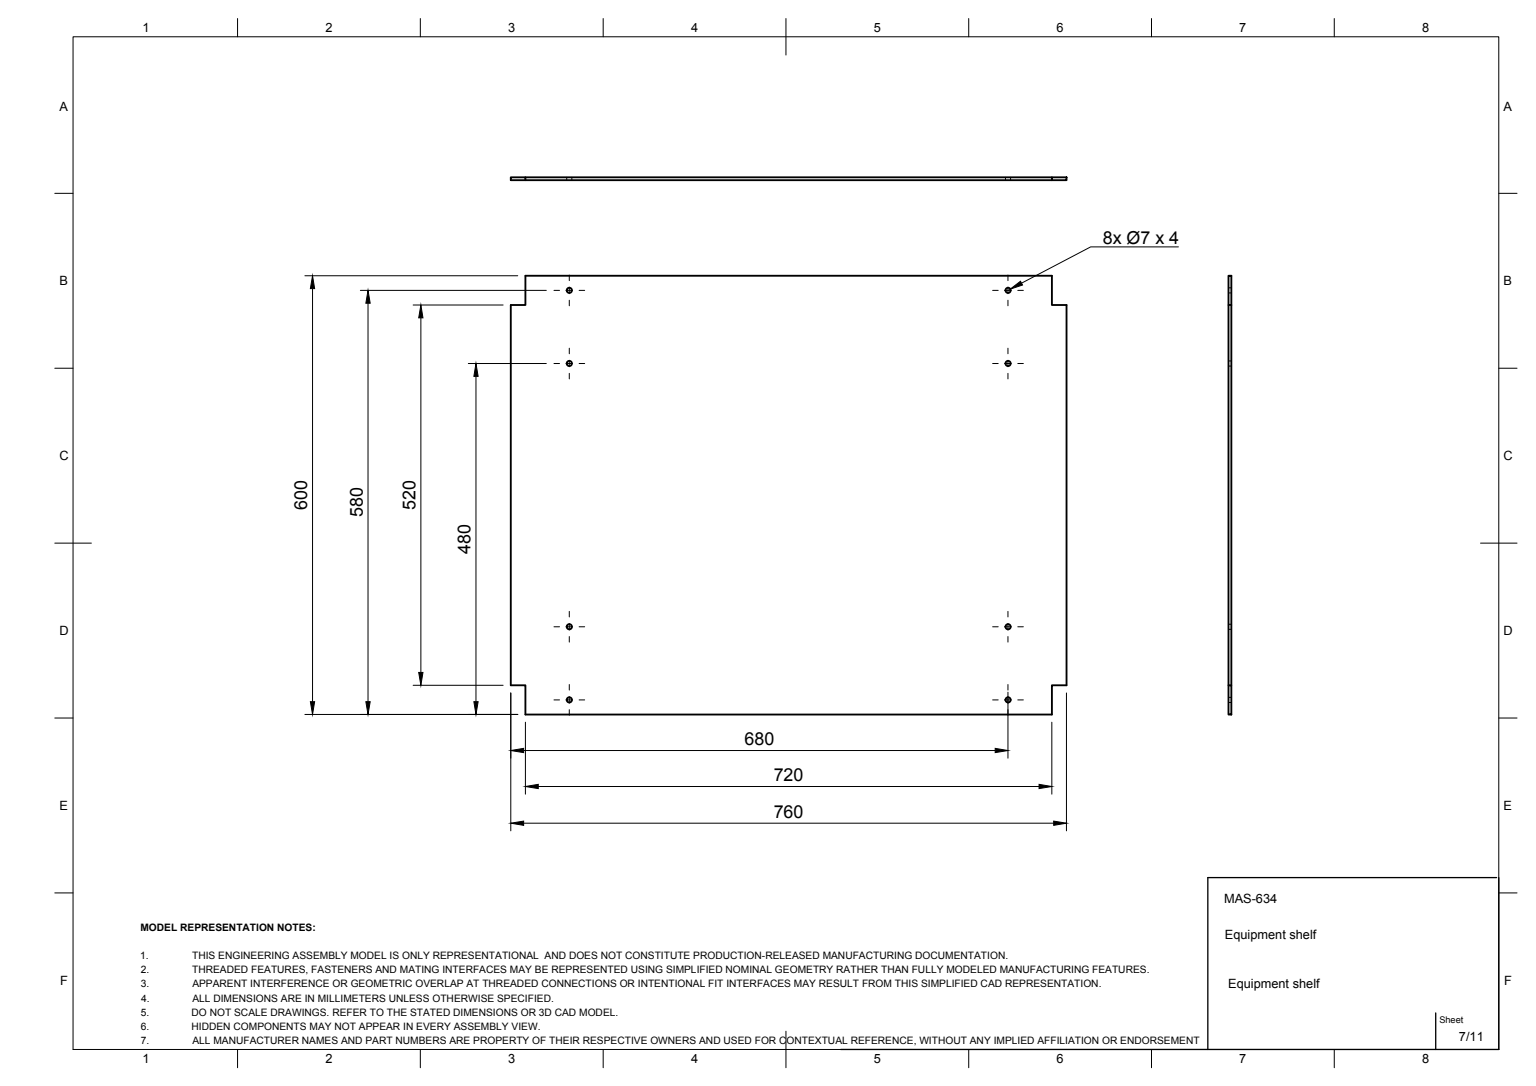
ISO-10303-21;
HEADER;
/* Generated by software containing ST-Developer
 * from STEP Tools, Inc. (www.steptools.com) 
 */

FILE_DESCRIPTION(
/* description */ ('Independent AHU equipment rack. Nominal800x600 frame on1000long40squa
re aluminum posts; two removable notched shelves; welded perimeter/cro
ss rails and rear gussets; two mounting channels; four isolation pads 
and anchor-ready feet. Imported native extrusion library retained and 
cut-length parameters customized per family. Shelf hardware uses model
ed M6 rivet nuts and screws. Weld design, floor anchors and load ratin
g require engineering selection.'),
/* implementation_level */ '2;1');

FILE_NAME(
/* name */ 'Equipment shelf.step',
/* time_stamp */ '2026-11-07T19:04:45-08:00',
/* author */ (''),
/* organization */ (''),
/* preprocessor_version */ 'ST-DEVELOPER v20.2',
/* originating_system */ 'Autodesk Translation Framework v15.17.0.0',
/* authorisation */ '');

FILE_SCHEMA (('AUTOMOTIVE_DESIGN { 1 0 10303 214 3 1 1 }'));
ENDSEC;

DATA;
#10=MECHANICAL_DESIGN_GEOMETRIC_PRESENTATION_REPRESENTATION('',(#339),#9777);
#317=SHAPE_REPRESENTATION_RELATIONSHIP('SRR','None',#9861,#328);
#328=ADVANCED_BREP_SHAPE_REPRESENTATION('',(#350),#9770);
#339=STYLED_ITEM('',(#9924),#350);
#350=MANIFOLD_SOLID_BREP('Body1',#3844);
#371=FACE_BOUND('',#809,.T.);
#372=FACE_BOUND('',#810,.T.);
#373=FACE_BOUND('',#811,.T.);
#374=FACE_BOUND('',#812,.T.);
#375=FACE_BOUND('',#813,.T.);
#376=FACE_BOUND('',#814,.T.);
#377=FACE_BOUND('',#815,.T.);
#378=FACE_BOUND('',#816,.T.);
#379=FACE_BOUND('',#818,.T.);
#380=FACE_BOUND('',#819,.T.);
#381=FACE_BOUND('',#820,.T.);
#382=FACE_BOUND('',#821,.T.);
#383=FACE_BOUND('',#822,.T.);
#384=FACE_BOUND('',#823,.T.);
#385=FACE_BOUND('',#824,.T.);
#386=FACE_BOUND('',#825,.T.);
#450=PLANE('',#4151);
#451=PLANE('',#4152);
#452=PLANE('',#4153);
#453=PLANE('',#4154);
#454=PLANE('',#4155);
#455=PLANE('',#4156);
#456=PLANE('',#4157);
#457=PLANE('',#4158);
#458=PLANE('',#4159);
#459=PLANE('',#4160);
#460=PLANE('',#4161);
#461=PLANE('',#4162);
#462=PLANE('',#4163);
#463=PLANE('',#4164);
#578=FACE_OUTER_BOUND('',#790,.T.);
#579=FACE_OUTER_BOUND('',#791,.T.);
#580=FACE_OUTER_BOUND('',#792,.T.);
#581=FACE_OUTER_BOUND('',#793,.T.);
#582=FACE_OUTER_BOUND('',#794,.T.);
#583=FACE_OUTER_BOUND('',#795,.T.);
#584=FACE_OUTER_BOUND('',#796,.T.);
#585=FACE_OUTER_BOUND('',#797,.T.);
#586=FACE_OUTER_BOUND('',#798,.T.);
#587=FACE_OUTER_BOUND('',#799,.T.);
#588=FACE_OUTER_BOUND('',#800,.T.);
#589=FACE_OUTER_BOUND('',#801,.T.);
#590=FACE_OUTER_BOUND('',#802,.T.);
#591=FACE_OUTER_BOUND('',#803,.T.);
#592=FACE_OUTER_BOUND('',#804,.T.);
#593=FACE_OUTER_BOUND('',#805,.T.);
#594=FACE_OUTER_BOUND('',#806,.T.);
#595=FACE_OUTER_BOUND('',#807,.T.);
#596=FACE_OUTER_BOUND('',#808,.T.);
#597=FACE_OUTER_BOUND('',#817,.T.);
#598=FACE_OUTER_BOUND('',#826,.T.);
#599=FACE_OUTER_BOUND('',#827,.T.);
#790=EDGE_LOOP('',(#2923,#2924,#2925,#2926));
#791=EDGE_LOOP('',(#2927,#2928,#2929,#2930));
#792=EDGE_LOOP('',(#2931,#2932,#2933,#2934));
#793=EDGE_LOOP('',(#2935,#2936,#2937,#2938));
#794=EDGE_LOOP('',(#2939,#2940,#2941,#2942));
#795=EDGE_LOOP('',(#2943,#2944,#2945,#2946));
#796=EDGE_LOOP('',(#2947,#2948,#2949,#2950));
#797=EDGE_LOOP('',(#2951,#2952,#2953,#2954));
#798=EDGE_LOOP('',(#2955,#2956,#2957,#2958));
#799=EDGE_LOOP('',(#2959,#2960,#2961,#2962));
#800=EDGE_LOOP('',(#2963,#2964,#2965,#2966));
#801=EDGE_LOOP('',(#2967,#2968,#2969,#2970));
#802=EDGE_LOOP('',(#2971,#2972,#2973,#2974));
#803=EDGE_LOOP('',(#2975,#2976,#2977,#2978));
#804=EDGE_LOOP('',(#2979,#2980,#2981,#2982));
#805=EDGE_LOOP('',(#2983,#2984,#2985,#2986));
#806=EDGE_LOOP('',(#2987,#2988,#2989,#2990));
#807=EDGE_LOOP('',(#2991,#2992,#2993,#2994));
#808=EDGE_LOOP('',(#2995,#2996,#2997,#2998,#2999,#3000,#3001,#3002,#3003,
#3004,#3005,#3006));
#809=EDGE_LOOP('',(#3007));
#810=EDGE_LOOP('',(#3008));
#811=EDGE_LOOP('',(#3009));
#812=EDGE_LOOP('',(#3010));
#813=EDGE_LOOP('',(#3011));
#814=EDGE_LOOP('',(#3012));
#815=EDGE_LOOP('',(#3013));
#816=EDGE_LOOP('',(#3014));
#817=EDGE_LOOP('',(#3015,#3016,#3017,#3018,#3019,#3020,#3021,#3022,#3023,
#3024,#3025,#3026));
#818=EDGE_LOOP('',(#3027));
#819=EDGE_LOOP('',(#3028));
#820=EDGE_LOOP('',(#3029));
#821=EDGE_LOOP('',(#3030));
#822=EDGE_LOOP('',(#3031));
#823=EDGE_LOOP('',(#3032));
#824=EDGE_LOOP('',(#3033));
#825=EDGE_LOOP('',(#3034));
#826=EDGE_LOOP('',(#3035,#3036,#3037,#3038));
#827=EDGE_LOOP('',(#3039,#3040,#3041,#3042));
#1083=LINE('',#5829,#1376);
#1084=LINE('',#5835,#1377);
#1085=LINE('',#5841,#1378);
#1086=LINE('',#5847,#1379);
#1087=LINE('',#5853,#1380);
#1088=LINE('',#5859,#1381);
#1089=LINE('',#5865,#1382);
#1090=LINE('',#5871,#1383);
#1091=LINE('',#5876,#1384);
#1092=LINE('',#5878,#1385);
#1093=LINE('',#5880,#1386);
#1094=LINE('',#5881,#1387);
#1095=LINE('',#5884,#1388);
#1096=LINE('',#5886,#1389);
#1097=LINE('',#5887,#1390);
#1098=LINE('',#5891,#1391);
#1099=LINE('',#5893,#1392);
#1100=LINE('',#5895,#1393);
#1101=LINE('',#5896,#1394);
#1102=LINE('',#5899,#1395);
#1103=LINE('',#5901,#1396);
#1104=LINE('',#5902,#1397);
#1105=LINE('',#5906,#1398);
#1106=LINE('',#5908,#1399);
#1107=LINE('',#5910,#1400);
#1108=LINE('',#5911,#1401);
#1109=LINE('',#5914,#1402);
#1110=LINE('',#5916,#1403);
#1111=LINE('',#5917,#1404);
#1112=LINE('',#5921,#1405);
#1113=LINE('',#5923,#1406);
#1114=LINE('',#5925,#1407);
#1115=LINE('',#5926,#1408);
#1116=LINE('',#5929,#1409);
#1117=LINE('',#5931,#1410);
#1118=LINE('',#5932,#1411);
#1119=LINE('',#5934,#1412);
#1120=LINE('',#5935,#1413);
#1121=LINE('',#5937,#1414);
#1122=LINE('',#5938,#1415);
#1123=LINE('',#5940,#1416);
#1124=LINE('',#5941,#1417);
#1125=LINE('',#5943,#1418);
#1126=LINE('',#5944,#1419);
#1376=VECTOR('',#4796,3.5);
#1377=VECTOR('',#4803,3.5);
#1378=VECTOR('',#4810,3.5);
#1379=VECTOR('',#4817,3.5);
#1380=VECTOR('',#4824,3.5);
#1381=VECTOR('',#4831,3.5);
#1382=VECTOR('',#4838,3.5);
#1383=VECTOR('',#4845,3.5);
#1384=VECTOR('',#4850,10.);
#1385=VECTOR('',#4851,10.);
#1386=VECTOR('',#4852,10.);
#1387=VECTOR('',#4853,10.);
#1388=VECTOR('',#4856,10.);
#1389=VECTOR('',#4857,10.);
#1390=VECTOR('',#4858,10.);
#1391=VECTOR('',#4861,10.);
#1392=VECTOR('',#4862,10.);
#1393=VECTOR('',#4863,10.);
#1394=VECTOR('',#4864,10.);
#1395=VECTOR('',#4867,10.);
#1396=VECTOR('',#4868,10.);
#1397=VECTOR('',#4869,10.);
#1398=VECTOR('',#4872,10.);
#1399=VECTOR('',#4873,10.);
#1400=VECTOR('',#4874,10.);
#1401=VECTOR('',#4875,10.);
#1402=VECTOR('',#4878,10.);
#1403=VECTOR('',#4879,10.);
#1404=VECTOR('',#4880,10.);
#1405=VECTOR('',#4883,10.);
#1406=VECTOR('',#4884,10.);
#1407=VECTOR('',#4885,10.);
#1408=VECTOR('',#4886,10.);
#1409=VECTOR('',#4889,10.);
#1410=VECTOR('',#4890,10.);
#1411=VECTOR('',#4891,10.);
#1412=VECTOR('',#4894,10.);
#1413=VECTOR('',#4895,10.);
#1414=VECTOR('',#4898,10.);
#1415=VECTOR('',#4899,10.);
#1416=VECTOR('',#4902,10.);
#1417=VECTOR('',#4903,10.);
#1418=VECTOR('',#4906,10.);
#1419=VECTOR('',#4907,10.);
#1609=CIRCLE('',#4128,3.5);
#1610=CIRCLE('',#4129,3.5);
#1611=CIRCLE('',#4131,3.5);
#1612=CIRCLE('',#4132,3.5);
#1613=CIRCLE('',#4134,3.5);
#1614=CIRCLE('',#4135,3.5);
#1615=CIRCLE('',#4137,3.5);
#1616=CIRCLE('',#4138,3.5);
#1617=CIRCLE('',#4140,3.5);
#1618=CIRCLE('',#4141,3.5);
#1619=CIRCLE('',#4143,3.5);
#1620=CIRCLE('',#4144,3.5);
#1621=CIRCLE('',#4146,3.5);
#1622=CIRCLE('',#4147,3.5);
#1623=CIRCLE('',#4149,3.5);
#1624=CIRCLE('',#4150,3.5);
#1796=VERTEX_POINT('',#5826);
#1797=VERTEX_POINT('',#5828);
#1798=VERTEX_POINT('',#5832);
#1799=VERTEX_POINT('',#5834);
#1800=VERTEX_POINT('',#5838);
#1801=VERTEX_POINT('',#5840);
#1802=VERTEX_POINT('',#5844);
#1803=VERTEX_POINT('',#5846);
#1804=VERTEX_POINT('',#5850);
#1805=VERTEX_POINT('',#5852);
#1806=VERTEX_POINT('',#5856);
#1807=VERTEX_POINT('',#5858);
#1808=VERTEX_POINT('',#5862);
#1809=VERTEX_POINT('',#5864);
#1810=VERTEX_POINT('',#5868);
#1811=VERTEX_POINT('',#5870);
#1812=VERTEX_POINT('',#5874);
#1813=VERTEX_POINT('',#5875);
#1814=VERTEX_POINT('',#5877);
#1815=VERTEX_POINT('',#5879);
#1816=VERTEX_POINT('',#5883);
#1817=VERTEX_POINT('',#5885);
#1818=VERTEX_POINT('',#5889);
#1819=VERTEX_POINT('',#5890);
#1820=VERTEX_POINT('',#5892);
#1821=VERTEX_POINT('',#5894);
#1822=VERTEX_POINT('',#5898);
#1823=VERTEX_POINT('',#5900);
#1824=VERTEX_POINT('',#5904);
#1825=VERTEX_POINT('',#5905);
#1826=VERTEX_POINT('',#5907);
#1827=VERTEX_POINT('',#5909);
#1828=VERTEX_POINT('',#5913);
#1829=VERTEX_POINT('',#5915);
#1830=VERTEX_POINT('',#5919);
#1831=VERTEX_POINT('',#5920);
#1832=VERTEX_POINT('',#5922);
#1833=VERTEX_POINT('',#5924);
#1834=VERTEX_POINT('',#5928);
#1835=VERTEX_POINT('',#5930);
#2206=EDGE_CURVE('',#1796,#1796,#1609,.T.);
#2207=EDGE_CURVE('',#1796,#1797,#1083,.T.);
#2208=EDGE_CURVE('',#1797,#1797,#1610,.T.);
#2209=EDGE_CURVE('',#1798,#1798,#1611,.T.);
#2210=EDGE_CURVE('',#1798,#1799,#1084,.T.);
#2211=EDGE_CURVE('',#1799,#1799,#1612,.T.);
#2212=EDGE_CURVE('',#1800,#1800,#1613,.T.);
#2213=EDGE_CURVE('',#1800,#1801,#1085,.T.);
#2214=EDGE_CURVE('',#1801,#1801,#1614,.T.);
#2215=EDGE_CURVE('',#1802,#1802,#1615,.T.);
#2216=EDGE_CURVE('',#1802,#1803,#1086,.T.);
#2217=EDGE_CURVE('',#1803,#1803,#1616,.T.);
#2218=EDGE_CURVE('',#1804,#1804,#1617,.T.);
#2219=EDGE_CURVE('',#1804,#1805,#1087,.T.);
#2220=EDGE_CURVE('',#1805,#1805,#1618,.T.);
#2221=EDGE_CURVE('',#1806,#1806,#1619,.T.);
#2222=EDGE_CURVE('',#1806,#1807,#1088,.T.);
#2223=EDGE_CURVE('',#1807,#1807,#1620,.T.);
#2224=EDGE_CURVE('',#1808,#1808,#1621,.T.);
#2225=EDGE_CURVE('',#1808,#1809,#1089,.T.);
#2226=EDGE_CURVE('',#1809,#1809,#1622,.T.);
#2227=EDGE_CURVE('',#1810,#1810,#1623,.T.);
#2228=EDGE_CURVE('',#1810,#1811,#1090,.T.);
#2229=EDGE_CURVE('',#1811,#1811,#1624,.T.);
#2230=EDGE_CURVE('',#1812,#1813,#1091,.T.);
#2231=EDGE_CURVE('',#1812,#1814,#1092,.T.);
#2232=EDGE_CURVE('',#1815,#1814,#1093,.T.);
#2233=EDGE_CURVE('',#1813,#1815,#1094,.T.);
#2234=EDGE_CURVE('',#1816,#1812,#1095,.T.);
#2235=EDGE_CURVE('',#1817,#1816,#1096,.T.);
#2236=EDGE_CURVE('',#1814,#1817,#1097,.T.);
#2237=EDGE_CURVE('',#1818,#1819,#1098,.T.);
#2238=EDGE_CURVE('',#1818,#1820,#1099,.T.);
#2239=EDGE_CURVE('',#1821,#1820,#1100,.T.);
#2240=EDGE_CURVE('',#1819,#1821,#1101,.T.);
#2241=EDGE_CURVE('',#1822,#1818,#1102,.T.);
#2242=EDGE_CURVE('',#1823,#1822,#1103,.T.);
#2243=EDGE_CURVE('',#1820,#1823,#1104,.T.);
#2244=EDGE_CURVE('',#1824,#1825,#1105,.T.);
#2245=EDGE_CURVE('',#1824,#1826,#1106,.T.);
#2246=EDGE_CURVE('',#1827,#1826,#1107,.T.);
#2247=EDGE_CURVE('',#1825,#1827,#1108,.T.);
#2248=EDGE_CURVE('',#1828,#1824,#1109,.T.);
#2249=EDGE_CURVE('',#1829,#1828,#1110,.T.);
#2250=EDGE_CURVE('',#1826,#1829,#1111,.T.);
#2251=EDGE_CURVE('',#1830,#1831,#1112,.T.);
#2252=EDGE_CURVE('',#1832,#1830,#1113,.T.);
#2253=EDGE_CURVE('',#1833,#1832,#1114,.T.);
#2254=EDGE_CURVE('',#1831,#1833,#1115,.T.);
#2255=EDGE_CURVE('',#1831,#1834,#1116,.T.);
#2256=EDGE_CURVE('',#1835,#1833,#1117,.T.);
#2257=EDGE_CURVE('',#1834,#1835,#1118,.T.);
#2258=EDGE_CURVE('',#1821,#1829,#1119,.T.);
#2259=EDGE_CURVE('',#1819,#1828,#1120,.T.);
#2260=EDGE_CURVE('',#1834,#1822,#1121,.T.);
#2261=EDGE_CURVE('',#1835,#1823,#1122,.T.);
#2262=EDGE_CURVE('',#1827,#1817,#1123,.T.);
#2263=EDGE_CURVE('',#1815,#1832,#1124,.T.);
#2264=EDGE_CURVE('',#1813,#1830,#1125,.T.);
#2265=EDGE_CURVE('',#1825,#1816,#1126,.T.);
#2923=ORIENTED_EDGE('',*,*,#2206,.F.);
#2924=ORIENTED_EDGE('',*,*,#2207,.T.);
#2925=ORIENTED_EDGE('',*,*,#2208,.F.);
#2926=ORIENTED_EDGE('',*,*,#2207,.F.);
#2927=ORIENTED_EDGE('',*,*,#2209,.F.);
#2928=ORIENTED_EDGE('',*,*,#2210,.T.);
#2929=ORIENTED_EDGE('',*,*,#2211,.F.);
#2930=ORIENTED_EDGE('',*,*,#2210,.F.);
#2931=ORIENTED_EDGE('',*,*,#2212,.F.);
#2932=ORIENTED_EDGE('',*,*,#2213,.T.);
#2933=ORIENTED_EDGE('',*,*,#2214,.F.);
#2934=ORIENTED_EDGE('',*,*,#2213,.F.);
#2935=ORIENTED_EDGE('',*,*,#2215,.F.);
#2936=ORIENTED_EDGE('',*,*,#2216,.T.);
#2937=ORIENTED_EDGE('',*,*,#2217,.F.);
#2938=ORIENTED_EDGE('',*,*,#2216,.F.);
#2939=ORIENTED_EDGE('',*,*,#2218,.F.);
#2940=ORIENTED_EDGE('',*,*,#2219,.T.);
#2941=ORIENTED_EDGE('',*,*,#2220,.F.);
#2942=ORIENTED_EDGE('',*,*,#2219,.F.);
#2943=ORIENTED_EDGE('',*,*,#2221,.F.);
#2944=ORIENTED_EDGE('',*,*,#2222,.T.);
#2945=ORIENTED_EDGE('',*,*,#2223,.F.);
#2946=ORIENTED_EDGE('',*,*,#2222,.F.);
#2947=ORIENTED_EDGE('',*,*,#2224,.F.);
#2948=ORIENTED_EDGE('',*,*,#2225,.T.);
#2949=ORIENTED_EDGE('',*,*,#2226,.F.);
#2950=ORIENTED_EDGE('',*,*,#2225,.F.);
#2951=ORIENTED_EDGE('',*,*,#2227,.F.);
#2952=ORIENTED_EDGE('',*,*,#2228,.T.);
#2953=ORIENTED_EDGE('',*,*,#2229,.F.);
#2954=ORIENTED_EDGE('',*,*,#2228,.F.);
#2955=ORIENTED_EDGE('',*,*,#2230,.F.);
#2956=ORIENTED_EDGE('',*,*,#2231,.T.);
#2957=ORIENTED_EDGE('',*,*,#2232,.F.);
#2958=ORIENTED_EDGE('',*,*,#2233,.F.);
#2959=ORIENTED_EDGE('',*,*,#2234,.F.);
#2960=ORIENTED_EDGE('',*,*,#2235,.F.);
#2961=ORIENTED_EDGE('',*,*,#2236,.F.);
#2962=ORIENTED_EDGE('',*,*,#2231,.F.);
#2963=ORIENTED_EDGE('',*,*,#2237,.F.);
#2964=ORIENTED_EDGE('',*,*,#2238,.T.);
#2965=ORIENTED_EDGE('',*,*,#2239,.F.);
#2966=ORIENTED_EDGE('',*,*,#2240,.F.);
#2967=ORIENTED_EDGE('',*,*,#2241,.F.);
#2968=ORIENTED_EDGE('',*,*,#2242,.F.);
#2969=ORIENTED_EDGE('',*,*,#2243,.F.);
#2970=ORIENTED_EDGE('',*,*,#2238,.F.);
#2971=ORIENTED_EDGE('',*,*,#2244,.F.);
#2972=ORIENTED_EDGE('',*,*,#2245,.T.);
#2973=ORIENTED_EDGE('',*,*,#2246,.F.);
#2974=ORIENTED_EDGE('',*,*,#2247,.F.);
#2975=ORIENTED_EDGE('',*,*,#2248,.F.);
#2976=ORIENTED_EDGE('',*,*,#2249,.F.);
#2977=ORIENTED_EDGE('',*,*,#2250,.F.);
#2978=ORIENTED_EDGE('',*,*,#2245,.F.);
#2979=ORIENTED_EDGE('',*,*,#2251,.F.);
#2980=ORIENTED_EDGE('',*,*,#2252,.F.);
#2981=ORIENTED_EDGE('',*,*,#2253,.F.);
#2982=ORIENTED_EDGE('',*,*,#2254,.F.);
#2983=ORIENTED_EDGE('',*,*,#2255,.F.);
#2984=ORIENTED_EDGE('',*,*,#2254,.T.);
#2985=ORIENTED_EDGE('',*,*,#2256,.F.);
#2986=ORIENTED_EDGE('',*,*,#2257,.F.);
#2987=ORIENTED_EDGE('',*,*,#2240,.T.);
#2988=ORIENTED_EDGE('',*,*,#2258,.T.);
#2989=ORIENTED_EDGE('',*,*,#2249,.T.);
#2990=ORIENTED_EDGE('',*,*,#2259,.F.);
#2991=ORIENTED_EDGE('',*,*,#2242,.T.);
#2992=ORIENTED_EDGE('',*,*,#2260,.F.);
#2993=ORIENTED_EDGE('',*,*,#2257,.T.);
#2994=ORIENTED_EDGE('',*,*,#2261,.T.);
#2995=ORIENTED_EDGE('',*,*,#2232,.T.);
#2996=ORIENTED_EDGE('',*,*,#2236,.T.);
#2997=ORIENTED_EDGE('',*,*,#2262,.F.);
#2998=ORIENTED_EDGE('',*,*,#2246,.T.);
#2999=ORIENTED_EDGE('',*,*,#2250,.T.);
#3000=ORIENTED_EDGE('',*,*,#2258,.F.);
#3001=ORIENTED_EDGE('',*,*,#2239,.T.);
#3002=ORIENTED_EDGE('',*,*,#2243,.T.);
#3003=ORIENTED_EDGE('',*,*,#2261,.F.);
#3004=ORIENTED_EDGE('',*,*,#2256,.T.);
#3005=ORIENTED_EDGE('',*,*,#2253,.T.);
#3006=ORIENTED_EDGE('',*,*,#2263,.F.);
#3007=ORIENTED_EDGE('',*,*,#2229,.T.);
#3008=ORIENTED_EDGE('',*,*,#2226,.T.);
#3009=ORIENTED_EDGE('',*,*,#2223,.T.);
#3010=ORIENTED_EDGE('',*,*,#2220,.T.);
#3011=ORIENTED_EDGE('',*,*,#2217,.T.);
#3012=ORIENTED_EDGE('',*,*,#2214,.T.);
#3013=ORIENTED_EDGE('',*,*,#2211,.T.);
#3014=ORIENTED_EDGE('',*,*,#2208,.T.);
#3015=ORIENTED_EDGE('',*,*,#2234,.T.);
#3016=ORIENTED_EDGE('',*,*,#2230,.T.);
#3017=ORIENTED_EDGE('',*,*,#2264,.T.);
#3018=ORIENTED_EDGE('',*,*,#2251,.T.);
#3019=ORIENTED_EDGE('',*,*,#2255,.T.);
#3020=ORIENTED_EDGE('',*,*,#2260,.T.);
#3021=ORIENTED_EDGE('',*,*,#2241,.T.);
#3022=ORIENTED_EDGE('',*,*,#2237,.T.);
#3023=ORIENTED_EDGE('',*,*,#2259,.T.);
#3024=ORIENTED_EDGE('',*,*,#2248,.T.);
#3025=ORIENTED_EDGE('',*,*,#2244,.T.);
#3026=ORIENTED_EDGE('',*,*,#2265,.T.);
#3027=ORIENTED_EDGE('',*,*,#2227,.T.);
#3028=ORIENTED_EDGE('',*,*,#2224,.T.);
#3029=ORIENTED_EDGE('',*,*,#2221,.T.);
#3030=ORIENTED_EDGE('',*,*,#2218,.T.);
#3031=ORIENTED_EDGE('',*,*,#2215,.T.);
#3032=ORIENTED_EDGE('',*,*,#2212,.T.);
#3033=ORIENTED_EDGE('',*,*,#2209,.T.);
#3034=ORIENTED_EDGE('',*,*,#2206,.T.);
#3035=ORIENTED_EDGE('',*,*,#2233,.T.);
#3036=ORIENTED_EDGE('',*,*,#2263,.T.);
#3037=ORIENTED_EDGE('',*,*,#2252,.T.);
#3038=ORIENTED_EDGE('',*,*,#2264,.F.);
#3039=ORIENTED_EDGE('',*,*,#2235,.T.);
#3040=ORIENTED_EDGE('',*,*,#2265,.F.);
#3041=ORIENTED_EDGE('',*,*,#2247,.T.);
#3042=ORIENTED_EDGE('',*,*,#2262,.T.);
#3577=CYLINDRICAL_SURFACE('',#4127,3.5);
#3578=CYLINDRICAL_SURFACE('',#4130,3.5);
#3579=CYLINDRICAL_SURFACE('',#4133,3.5);
#3580=CYLINDRICAL_SURFACE('',#4136,3.5);
#3581=CYLINDRICAL_SURFACE('',#4139,3.5);
#3582=CYLINDRICAL_SURFACE('',#4142,3.5);
#3583=CYLINDRICAL_SURFACE('',#4145,3.5);
#3584=CYLINDRICAL_SURFACE('',#4148,3.5);
#3718=ADVANCED_FACE('',(#578),#3577,.F.);
#3719=ADVANCED_FACE('',(#579),#3578,.F.);
#3720=ADVANCED_FACE('',(#580),#3579,.F.);
#3721=ADVANCED_FACE('',(#581),#3580,.F.);
#3722=ADVANCED_FACE('',(#582),#3581,.F.);
#3723=ADVANCED_FACE('',(#583),#3582,.F.);
#3724=ADVANCED_FACE('',(#584),#3583,.F.);
#3725=ADVANCED_FACE('',(#585),#3584,.F.);
#3726=ADVANCED_FACE('',(#586),#450,.F.);
#3727=ADVANCED_FACE('',(#587),#451,.F.);
#3728=ADVANCED_FACE('',(#588),#452,.F.);
#3729=ADVANCED_FACE('',(#589),#453,.F.);
#3730=ADVANCED_FACE('',(#590),#454,.F.);
#3731=ADVANCED_FACE('',(#591),#455,.F.);
#3732=ADVANCED_FACE('',(#592),#456,.F.);
#3733=ADVANCED_FACE('',(#593),#457,.F.);
#3734=ADVANCED_FACE('',(#594),#458,.T.);
#3735=ADVANCED_FACE('',(#595),#459,.T.);
#3736=ADVANCED_FACE('',(#596,#371,#372,#373,#374,#375,#376,#377,#378),#460,
 .F.);
#3737=ADVANCED_FACE('',(#597,#379,#380,#381,#382,#383,#384,#385,#386),#461,
 .T.);
#3738=ADVANCED_FACE('',(#598),#462,.T.);
#3739=ADVANCED_FACE('',(#599),#463,.T.);
#3844=CLOSED_SHELL('',(#3718,#3719,#3720,#3721,#3722,#3723,#3724,#3725,
#3726,#3727,#3728,#3729,#3730,#3731,#3732,#3733,#3734,#3735,#3736,#3737,
#3738,#3739));
#4126=AXIS2_PLACEMENT_3D('',#5824,#4790,#4791);
#4127=AXIS2_PLACEMENT_3D('',#5825,#4792,#4793);
#4128=AXIS2_PLACEMENT_3D('',#5827,#4794,#4795);
#4129=AXIS2_PLACEMENT_3D('',#5830,#4797,#4798);
#4130=AXIS2_PLACEMENT_3D('',#5831,#4799,#4800);
#4131=AXIS2_PLACEMENT_3D('',#5833,#4801,#4802);
#4132=AXIS2_PLACEMENT_3D('',#5836,#4804,#4805);
#4133=AXIS2_PLACEMENT_3D('',#5837,#4806,#4807);
#4134=AXIS2_PLACEMENT_3D('',#5839,#4808,#4809);
#4135=AXIS2_PLACEMENT_3D('',#5842,#4811,#4812);
#4136=AXIS2_PLACEMENT_3D('',#5843,#4813,#4814);
#4137=AXIS2_PLACEMENT_3D('',#5845,#4815,#4816);
#4138=AXIS2_PLACEMENT_3D('',#5848,#4818,#4819);
#4139=AXIS2_PLACEMENT_3D('',#5849,#4820,#4821);
#4140=AXIS2_PLACEMENT_3D('',#5851,#4822,#4823);
#4141=AXIS2_PLACEMENT_3D('',#5854,#4825,#4826);
#4142=AXIS2_PLACEMENT_3D('',#5855,#4827,#4828);
#4143=AXIS2_PLACEMENT_3D('',#5857,#4829,#4830);
#4144=AXIS2_PLACEMENT_3D('',#5860,#4832,#4833);
#4145=AXIS2_PLACEMENT_3D('',#5861,#4834,#4835);
#4146=AXIS2_PLACEMENT_3D('',#5863,#4836,#4837);
#4147=AXIS2_PLACEMENT_3D('',#5866,#4839,#4840);
#4148=AXIS2_PLACEMENT_3D('',#5867,#4841,#4842);
#4149=AXIS2_PLACEMENT_3D('',#5869,#4843,#4844);
#4150=AXIS2_PLACEMENT_3D('',#5872,#4846,#4847);
#4151=AXIS2_PLACEMENT_3D('',#5873,#4848,#4849);
#4152=AXIS2_PLACEMENT_3D('',#5882,#4854,#4855);
#4153=AXIS2_PLACEMENT_3D('',#5888,#4859,#4860);
#4154=AXIS2_PLACEMENT_3D('',#5897,#4865,#4866);
#4155=AXIS2_PLACEMENT_3D('',#5903,#4870,#4871);
#4156=AXIS2_PLACEMENT_3D('',#5912,#4876,#4877);
#4157=AXIS2_PLACEMENT_3D('',#5918,#4881,#4882);
#4158=AXIS2_PLACEMENT_3D('',#5927,#4887,#4888);
#4159=AXIS2_PLACEMENT_3D('',#5933,#4892,#4893);
#4160=AXIS2_PLACEMENT_3D('',#5936,#4896,#4897);
#4161=AXIS2_PLACEMENT_3D('',#5939,#4900,#4901);
#4162=AXIS2_PLACEMENT_3D('',#5942,#4904,#4905);
#4163=AXIS2_PLACEMENT_3D('',#5945,#4908,#4909);
#4164=AXIS2_PLACEMENT_3D('',#5946,#4910,#4911);
#4790=DIRECTION('axis',(0.,0.,1.));
#4791=DIRECTION('refdir',(1.,0.,0.));
#4792=DIRECTION('center_axis',(0.,0.,-1.));
#4793=DIRECTION('ref_axis',(1.,0.,0.));
#4794=DIRECTION('center_axis',(0.,0.,-1.));
#4795=DIRECTION('ref_axis',(1.,0.,0.));
#4796=DIRECTION('',(0.,0.,-1.));
#4797=DIRECTION('center_axis',(0.,0.,1.));
#4798=DIRECTION('ref_axis',(1.,0.,0.));
#4799=DIRECTION('center_axis',(0.,0.,-1.));
#4800=DIRECTION('ref_axis',(1.,0.,0.));
#4801=DIRECTION('center_axis',(0.,0.,-1.));
#4802=DIRECTION('ref_axis',(1.,0.,0.));
#4803=DIRECTION('',(0.,0.,-1.));
#4804=DIRECTION('center_axis',(0.,0.,1.));
#4805=DIRECTION('ref_axis',(1.,0.,0.));
#4806=DIRECTION('center_axis',(0.,0.,-1.));
#4807=DIRECTION('ref_axis',(1.,0.,0.));
#4808=DIRECTION('center_axis',(0.,0.,-1.));
#4809=DIRECTION('ref_axis',(1.,0.,0.));
#4810=DIRECTION('',(0.,0.,-1.));
#4811=DIRECTION('center_axis',(0.,0.,1.));
#4812=DIRECTION('ref_axis',(1.,0.,0.));
#4813=DIRECTION('center_axis',(0.,0.,-1.));
#4814=DIRECTION('ref_axis',(1.,0.,0.));
#4815=DIRECTION('center_axis',(0.,0.,-1.));
#4816=DIRECTION('ref_axis',(1.,0.,0.));
#4817=DIRECTION('',(0.,0.,-1.));
#4818=DIRECTION('center_axis',(0.,0.,1.));
#4819=DIRECTION('ref_axis',(1.,0.,0.));
#4820=DIRECTION('center_axis',(0.,0.,-1.));
#4821=DIRECTION('ref_axis',(1.,0.,0.));
#4822=DIRECTION('center_axis',(0.,0.,-1.));
#4823=DIRECTION('ref_axis',(1.,0.,0.));
#4824=DIRECTION('',(0.,0.,-1.));
#4825=DIRECTION('center_axis',(0.,0.,1.));
#4826=DIRECTION('ref_axis',(1.,0.,0.));
#4827=DIRECTION('center_axis',(0.,0.,-1.));
#4828=DIRECTION('ref_axis',(1.,0.,0.));
#4829=DIRECTION('center_axis',(0.,0.,-1.));
#4830=DIRECTION('ref_axis',(1.,0.,0.));
#4831=DIRECTION('',(0.,0.,-1.));
#4832=DIRECTION('center_axis',(0.,0.,1.));
#4833=DIRECTION('ref_axis',(1.,0.,0.));
#4834=DIRECTION('center_axis',(0.,0.,-1.));
#4835=DIRECTION('ref_axis',(1.,0.,0.));
#4836=DIRECTION('center_axis',(0.,0.,-1.));
#4837=DIRECTION('ref_axis',(1.,0.,0.));
#4838=DIRECTION('',(0.,0.,-1.));
#4839=DIRECTION('center_axis',(0.,0.,1.));
#4840=DIRECTION('ref_axis',(1.,0.,0.));
#4841=DIRECTION('center_axis',(0.,0.,-1.));
#4842=DIRECTION('ref_axis',(1.,0.,0.));
#4843=DIRECTION('center_axis',(0.,0.,-1.));
#4844=DIRECTION('ref_axis',(1.,0.,0.));
#4845=DIRECTION('',(0.,0.,-1.));
#4846=DIRECTION('center_axis',(0.,0.,1.));
#4847=DIRECTION('ref_axis',(1.,0.,0.));
#4848=DIRECTION('center_axis',(0.,1.,0.));
#4849=DIRECTION('ref_axis',(1.,0.,0.));
#4850=DIRECTION('',(1.,0.,0.));
#4851=DIRECTION('',(0.,0.,-1.));
#4852=DIRECTION('',(-1.,0.,0.));
#4853=DIRECTION('',(0.,0.,-1.));
#4854=DIRECTION('center_axis',(-1.,0.,0.));
#4855=DIRECTION('ref_axis',(0.,1.,0.));
#4856=DIRECTION('',(0.,1.,0.));
#4857=DIRECTION('',(0.,0.,1.));
#4858=DIRECTION('',(0.,-1.,0.));
#4859=DIRECTION('center_axis',(0.,-1.,0.));
#4860=DIRECTION('ref_axis',(-1.,0.,0.));
#4861=DIRECTION('',(-1.,0.,0.));
#4862=DIRECTION('',(0.,0.,-1.));
#4863=DIRECTION('',(1.,0.,0.));
#4864=DIRECTION('',(0.,0.,-1.));
#4865=DIRECTION('center_axis',(1.,0.,0.));
#4866=DIRECTION('ref_axis',(0.,-1.,0.));
#4867=DIRECTION('',(0.,-1.,0.));
#4868=DIRECTION('',(0.,0.,1.));
#4869=DIRECTION('',(0.,1.,0.));
#4870=DIRECTION('center_axis',(1.,0.,0.));
#4871=DIRECTION('ref_axis',(0.,-1.,0.));
#4872=DIRECTION('',(0.,-1.,0.));
#4873=DIRECTION('',(0.,0.,-1.));
#4874=DIRECTION('',(0.,1.,0.));
#4875=DIRECTION('',(0.,0.,-1.));
#4876=DIRECTION('center_axis',(0.,1.,0.));
#4877=DIRECTION('ref_axis',(1.,0.,0.));
#4878=DIRECTION('',(1.,0.,0.));
#4879=DIRECTION('',(0.,0.,1.));
#4880=DIRECTION('',(-1.,0.,0.));
#4881=DIRECTION('center_axis',(0.,-1.,0.));
#4882=DIRECTION('ref_axis',(-1.,0.,0.));
#4883=DIRECTION('',(-1.,0.,0.));
#4884=DIRECTION('',(0.,0.,1.));
#4885=DIRECTION('',(1.,0.,0.));
#4886=DIRECTION('',(0.,0.,-1.));
#4887=DIRECTION('center_axis',(-1.,0.,0.));
#4888=DIRECTION('ref_axis',(0.,1.,0.));
#4889=DIRECTION('',(0.,1.,0.));
#4890=DIRECTION('',(0.,-1.,0.));
#4891=DIRECTION('',(0.,0.,-1.));
#4892=DIRECTION('center_axis',(-1.,0.,0.));
#4893=DIRECTION('ref_axis',(0.,-1.,0.));
#4894=DIRECTION('',(0.,-1.,0.));
#4895=DIRECTION('',(0.,-1.,0.));
#4896=DIRECTION('center_axis',(0.,1.,0.));
#4897=DIRECTION('ref_axis',(-1.,0.,0.));
#4898=DIRECTION('',(-1.,0.,0.));
#4899=DIRECTION('',(-1.,0.,0.));
#4900=DIRECTION('center_axis',(0.,0.,1.));
#4901=DIRECTION('ref_axis',(1.,0.,0.));
#4902=DIRECTION('',(1.,0.,0.));
#4903=DIRECTION('',(0.,1.,0.));
#4904=DIRECTION('center_axis',(0.,0.,1.));
#4905=DIRECTION('ref_axis',(1.,0.,0.));
#4906=DIRECTION('',(0.,1.,0.));
#4907=DIRECTION('',(1.,0.,0.));
#4908=DIRECTION('center_axis',(1.,0.,0.));
#4909=DIRECTION('ref_axis',(0.,1.,0.));
#4910=DIRECTION('center_axis',(0.,-1.,0.));
#4911=DIRECTION('ref_axis',(1.,0.,0.));
#5824=CARTESIAN_POINT('',(0.,0.,0.));
#5825=CARTESIAN_POINT('Origin',(300.,180.,2.));
#5826=CARTESIAN_POINT('',(296.5,180.,4.));
#5827=CARTESIAN_POINT('Origin',(300.,180.,4.));
#5828=CARTESIAN_POINT('',(296.5,180.,0.));
#5829=CARTESIAN_POINT('',(296.5,180.,2.));
#5830=CARTESIAN_POINT('Origin',(300.,180.,0.));
#5831=CARTESIAN_POINT('Origin',(300.,-280.,2.));
#5832=CARTESIAN_POINT('',(296.5,-280.,4.));
#5833=CARTESIAN_POINT('Origin',(300.,-280.,4.));
#5834=CARTESIAN_POINT('',(296.5,-280.,0.));
#5835=CARTESIAN_POINT('',(296.5,-280.,2.));
#5836=CARTESIAN_POINT('Origin',(300.,-280.,0.));
#5837=CARTESIAN_POINT('Origin',(-300.,180.,2.));
#5838=CARTESIAN_POINT('',(-303.5,180.,4.));
#5839=CARTESIAN_POINT('Origin',(-300.,180.,4.));
#5840=CARTESIAN_POINT('',(-303.5,180.,0.));
#5841=CARTESIAN_POINT('',(-303.5,180.,2.));
#5842=CARTESIAN_POINT('Origin',(-300.,180.,0.));
#5843=CARTESIAN_POINT('Origin',(-300.,-280.,2.));
#5844=CARTESIAN_POINT('',(-303.5,-280.,4.));
#5845=CARTESIAN_POINT('Origin',(-300.,-280.,4.));
#5846=CARTESIAN_POINT('',(-303.5,-280.,0.));
#5847=CARTESIAN_POINT('',(-303.5,-280.,2.));
#5848=CARTESIAN_POINT('Origin',(-300.,-280.,0.));
#5849=CARTESIAN_POINT('Origin',(-300.,-180.,2.));
#5850=CARTESIAN_POINT('',(-303.5,-180.,4.));
#5851=CARTESIAN_POINT('Origin',(-300.,-180.,4.));
#5852=CARTESIAN_POINT('',(-303.5,-180.,0.));
#5853=CARTESIAN_POINT('',(-303.5,-180.,2.));
#5854=CARTESIAN_POINT('Origin',(-300.,-180.,0.));
#5855=CARTESIAN_POINT('Origin',(-300.,280.,2.));
#5856=CARTESIAN_POINT('',(-303.5,280.,4.));
#5857=CARTESIAN_POINT('Origin',(-300.,280.,4.));
#5858=CARTESIAN_POINT('',(-303.5,280.,0.));
#5859=CARTESIAN_POINT('',(-303.5,280.,2.));
#5860=CARTESIAN_POINT('Origin',(-300.,280.,0.));
#5861=CARTESIAN_POINT('Origin',(300.,-180.,2.));
#5862=CARTESIAN_POINT('',(296.5,-180.,4.));
#5863=CARTESIAN_POINT('Origin',(300.,-180.,4.));
#5864=CARTESIAN_POINT('',(296.5,-180.,0.));
#5865=CARTESIAN_POINT('',(296.5,-180.,2.));
#5866=CARTESIAN_POINT('Origin',(300.,-180.,0.));
#5867=CARTESIAN_POINT('Origin',(300.,280.,2.));
#5868=CARTESIAN_POINT('',(296.5,280.,4.));
#5869=CARTESIAN_POINT('Origin',(300.,280.,4.));
#5870=CARTESIAN_POINT('',(296.5,280.,0.));
#5871=CARTESIAN_POINT('',(296.5,280.,2.));
#5872=CARTESIAN_POINT('Origin',(300.,280.,0.));
#5873=CARTESIAN_POINT('Origin',(360.,-260.,4.));
#5874=CARTESIAN_POINT('',(360.,-260.,4.));
#5875=CARTESIAN_POINT('',(380.,-260.,4.));
#5876=CARTESIAN_POINT('',(180.,-260.,4.));
#5877=CARTESIAN_POINT('',(360.,-260.,0.));
#5878=CARTESIAN_POINT('',(360.,-260.,4.));
#5879=CARTESIAN_POINT('',(380.,-260.,0.));
#5880=CARTESIAN_POINT('',(180.,-260.,0.));
#5881=CARTESIAN_POINT('',(380.,-260.,2.));
#5882=CARTESIAN_POINT('Origin',(360.,-300.,4.));
#5883=CARTESIAN_POINT('',(360.,-300.,4.));
#5884=CARTESIAN_POINT('',(360.,-150.,4.));
#5885=CARTESIAN_POINT('',(360.,-300.,0.));
#5886=CARTESIAN_POINT('',(360.,-300.,2.));
#5887=CARTESIAN_POINT('',(360.,-150.,0.));
#5888=CARTESIAN_POINT('Origin',(-360.,260.,4.));
#5889=CARTESIAN_POINT('',(-360.,260.,4.));
#5890=CARTESIAN_POINT('',(-380.,260.,4.));
#5891=CARTESIAN_POINT('',(-180.,260.,4.));
#5892=CARTESIAN_POINT('',(-360.,260.,0.));
#5893=CARTESIAN_POINT('',(-360.,260.,4.));
#5894=CARTESIAN_POINT('',(-380.,260.,0.));
#5895=CARTESIAN_POINT('',(-180.,260.,0.));
#5896=CARTESIAN_POINT('',(-380.,260.,2.));
#5897=CARTESIAN_POINT('Origin',(-360.,300.,4.));
#5898=CARTESIAN_POINT('',(-360.,300.,4.));
#5899=CARTESIAN_POINT('',(-360.,150.,4.));
#5900=CARTESIAN_POINT('',(-360.,300.,0.));
#5901=CARTESIAN_POINT('',(-360.,300.,2.));
#5902=CARTESIAN_POINT('',(-360.,150.,0.));
#5903=CARTESIAN_POINT('Origin',(-360.,-260.,4.));
#5904=CARTESIAN_POINT('',(-360.,-260.,4.));
#5905=CARTESIAN_POINT('',(-360.,-300.,4.));
#5906=CARTESIAN_POINT('',(-360.,-130.,4.));
#5907=CARTESIAN_POINT('',(-360.,-260.,0.));
#5908=CARTESIAN_POINT('',(-360.,-260.,4.));
#5909=CARTESIAN_POINT('',(-360.,-300.,0.));
#5910=CARTESIAN_POINT('',(-360.,-130.,0.));
#5911=CARTESIAN_POINT('',(-360.,-300.,2.));
#5912=CARTESIAN_POINT('Origin',(-380.,-260.,4.));
#5913=CARTESIAN_POINT('',(-380.,-260.,4.));
#5914=CARTESIAN_POINT('',(-190.,-260.,4.));
#5915=CARTESIAN_POINT('',(-380.,-260.,0.));
#5916=CARTESIAN_POINT('',(-380.,-260.,2.));
#5917=CARTESIAN_POINT('',(-190.,-260.,0.));
#5918=CARTESIAN_POINT('Origin',(380.,260.,4.));
#5919=CARTESIAN_POINT('',(380.,260.,4.));
#5920=CARTESIAN_POINT('',(360.,260.,4.));
#5921=CARTESIAN_POINT('',(190.,260.,4.));
#5922=CARTESIAN_POINT('',(380.,260.,0.));
#5923=CARTESIAN_POINT('',(380.,260.,2.));
#5924=CARTESIAN_POINT('',(360.,260.,0.));
#5925=CARTESIAN_POINT('',(190.,260.,0.));
#5926=CARTESIAN_POINT('',(360.,260.,4.));
#5927=CARTESIAN_POINT('Origin',(360.,260.,4.));
#5928=CARTESIAN_POINT('',(360.,300.,4.));
#5929=CARTESIAN_POINT('',(360.,130.,4.));
#5930=CARTESIAN_POINT('',(360.,300.,0.));
#5931=CARTESIAN_POINT('',(360.,130.,0.));
#5932=CARTESIAN_POINT('',(360.,300.,2.));
#5933=CARTESIAN_POINT('Origin',(-380.,300.,0.));
#5934=CARTESIAN_POINT('',(-380.,300.,0.));
#5935=CARTESIAN_POINT('',(-380.,300.,4.));
#5936=CARTESIAN_POINT('Origin',(380.,300.,0.));
#5937=CARTESIAN_POINT('',(380.,300.,4.));
#5938=CARTESIAN_POINT('',(380.,300.,0.));
#5939=CARTESIAN_POINT('Origin',(0.,0.,0.));
#5940=CARTESIAN_POINT('',(-380.,-300.,0.));
#5941=CARTESIAN_POINT('',(380.,-300.,0.));
#5942=CARTESIAN_POINT('Origin',(0.,0.,4.));
#5943=CARTESIAN_POINT('',(380.,-300.,4.));
#5944=CARTESIAN_POINT('',(-380.,-300.,4.));
#5945=CARTESIAN_POINT('Origin',(380.,-300.,0.));
#5946=CARTESIAN_POINT('Origin',(-380.,-300.,0.));
#9757=UNCERTAINTY_MEASURE_WITH_UNIT(LENGTH_MEASURE(0.01),#9778,
'DISTANCE_ACCURACY_VALUE',
'Maximum model space distance between geometric entities at asserted c
onnectivities');
#9764=UNCERTAINTY_MEASURE_WITH_UNIT(LENGTH_MEASURE(0.01),#9778,
'DISTANCE_ACCURACY_VALUE',
'Maximum model space distance between geometric entities at asserted c
onnectivities');
#9770=(
GEOMETRIC_REPRESENTATION_CONTEXT(3)
GLOBAL_UNCERTAINTY_ASSIGNED_CONTEXT((#9757))
GLOBAL_UNIT_ASSIGNED_CONTEXT((#9778,#9780,#9781))
REPRESENTATION_CONTEXT('','3D')
);
#9777=(
GEOMETRIC_REPRESENTATION_CONTEXT(3)
GLOBAL_UNCERTAINTY_ASSIGNED_CONTEXT((#9764))
GLOBAL_UNIT_ASSIGNED_CONTEXT((#9778,#9780,#9781))
REPRESENTATION_CONTEXT('','3D')
);
#9778=(
LENGTH_UNIT()
NAMED_UNIT(*)
SI_UNIT(.MILLI.,.METRE.)
);
#9780=(
NAMED_UNIT(*)
PLANE_ANGLE_UNIT()
SI_UNIT($,.RADIAN.)
);
#9781=(
NAMED_UNIT(*)
SI_UNIT($,.STERADIAN.)
SOLID_ANGLE_UNIT()
);
#9787=SHAPE_DEFINITION_REPRESENTATION(#9799,#9861);
#9799=PRODUCT_DEFINITION_SHAPE('',$,#9874);
#9861=SHAPE_REPRESENTATION('',(#4126),#9770);
#9868=PRODUCT_DEFINITION_CONTEXT('part definition',#9906,'design');
#9874=PRODUCT_DEFINITION('Equipment shelf','Equipment shelf',#9886,#9868);
#9886=PRODUCT_DEFINITION_FORMATION('',$,#9913);
#9906=APPLICATION_CONTEXT(
'Core Data for Automotive Mechanical Design Process');
#9907=PRODUCT_CONTEXT('part definition',#9906,'mechanical');
#9913=PRODUCT('Equipment shelf','Equipment shelf',$,(#9907));
#9924=PRESENTATION_STYLE_ASSIGNMENT((#9935));
#9935=SURFACE_STYLE_USAGE(.BOTH.,#9946);
#9946=SURFACE_SIDE_STYLE('',(#9957));
#9957=SURFACE_STYLE_FILL_AREA(#9968);
#9968=FILL_AREA_STYLE('Light blue',(#9979));
#9979=FILL_AREA_STYLE_COLOUR('Light blue',#9990);
#9990=COLOUR_RGB('Light blue',0.662745098039216,0.831372549019608,0.949019607843137);
ENDSEC;
END-ISO-10303-21;
